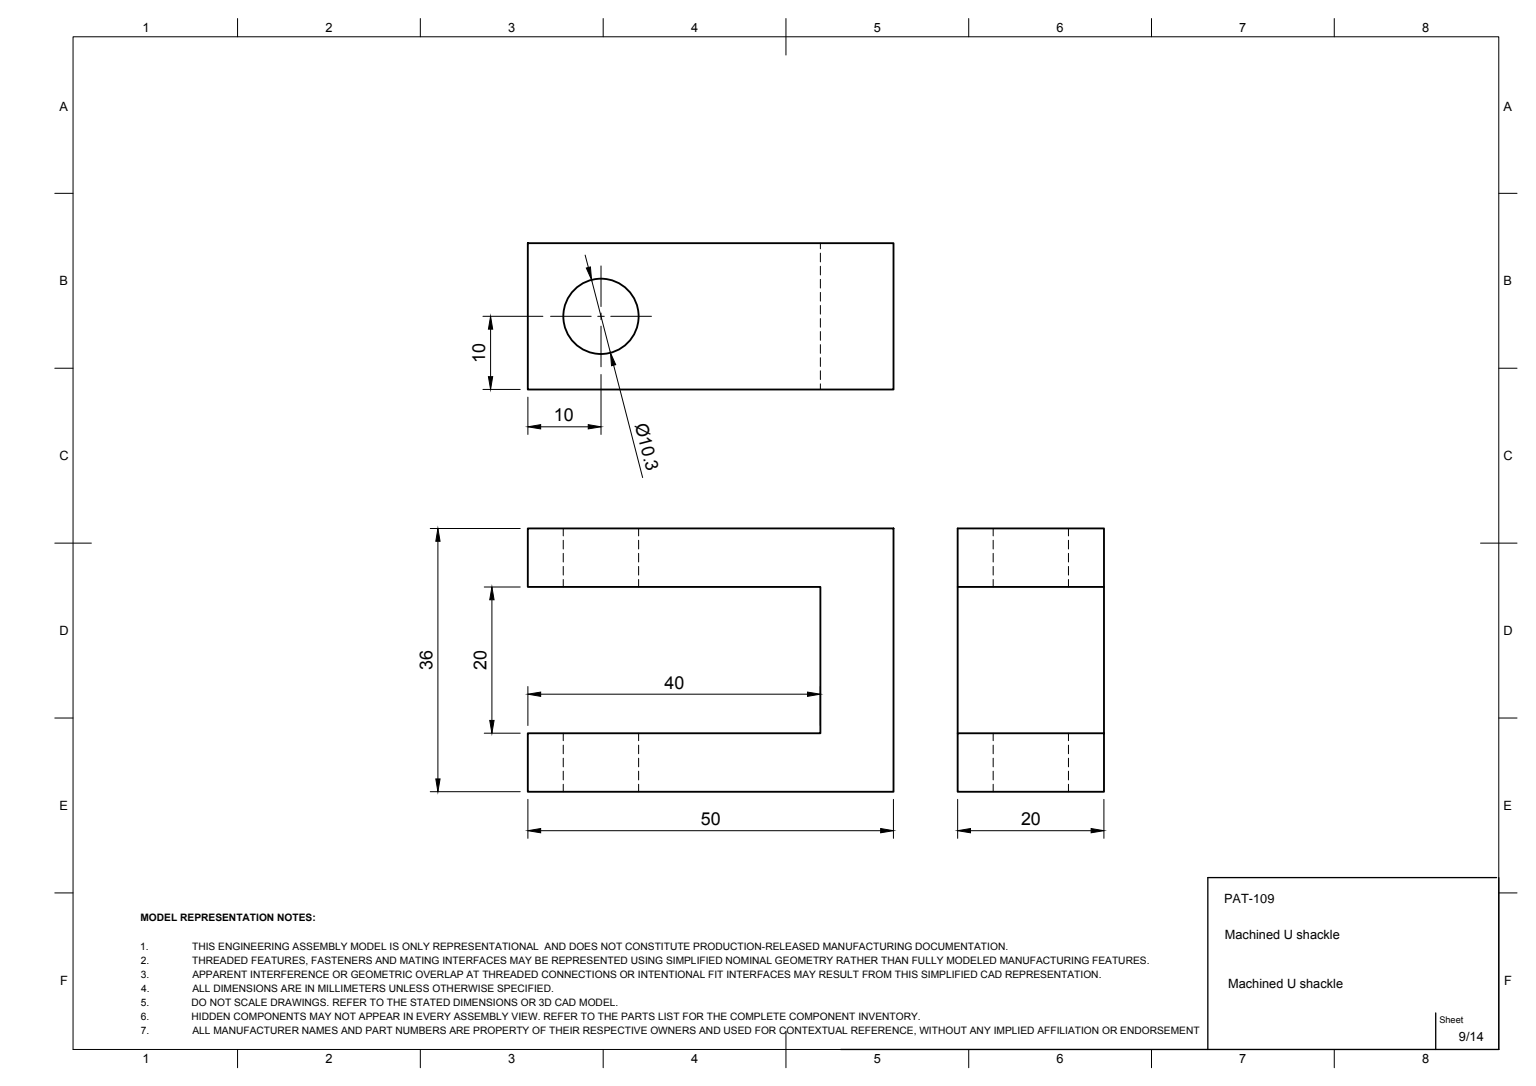
ISO-10303-21;
HEADER;
/* Generated by software containing ST-Developer
 * from STEP Tools, Inc. (www.steptools.com) 
 */

FILE_DESCRIPTION(
/* description */ ('Twin-shackle spreader bar'),
/* implementation_level */ '2;1');

FILE_NAME(
/* name */ 'Machined U shackle.step',
/* time_stamp */ '2026-10-27T20:18:10-07:00',
/* author */ (''),
/* organization */ (''),
/* preprocessor_version */ 'ST-DEVELOPER v20.2',
/* originating_system */ 'Autodesk Translation Framework v15.17.0.0',
/* authorisation */ '');

FILE_SCHEMA (('AUTOMOTIVE_DESIGN { 1 0 10303 214 3 1 1 }'));
ENDSEC;

DATA;
#10=MECHANICAL_DESIGN_GEOMETRIC_PRESENTATION_REPRESENTATION('',(#159),#1829);
#108=CIRCLE('',#1055,0.515000000000001);
#109=CIRCLE('',#1056,0.515000000000001);
#110=CIRCLE('',#1058,0.515000000000001);
#111=CIRCLE('',#1059,0.515000000000001);
#133=CYLINDRICAL_SURFACE('',#1054,0.515000000000001);
#134=CYLINDRICAL_SURFACE('',#1057,0.515000000000001);
#145=SHAPE_REPRESENTATION_RELATIONSHIP('SRR','None',#1883,#152);
#152=ADVANCED_BREP_SHAPE_REPRESENTATION('',(#166),#1824);
#159=STYLED_ITEM('',(#1970),#166);
#166=MANIFOLD_SOLID_BREP('Body1',#939);
#175=FACE_BOUND('',#260,.T.);
#176=FACE_BOUND('',#263,.T.);
#177=FACE_BOUND('',#266,.T.);
#178=FACE_BOUND('',#269,.T.);
#203=FACE_OUTER_BOUND('',#257,.T.);
#204=FACE_OUTER_BOUND('',#258,.T.);
#205=FACE_OUTER_BOUND('',#259,.T.);
#206=FACE_OUTER_BOUND('',#261,.T.);
#207=FACE_OUTER_BOUND('',#262,.T.);
#208=FACE_OUTER_BOUND('',#264,.T.);
#209=FACE_OUTER_BOUND('',#265,.T.);
#210=FACE_OUTER_BOUND('',#267,.T.);
#211=FACE_OUTER_BOUND('',#268,.T.);
#212=FACE_OUTER_BOUND('',#270,.T.);
#213=FACE_OUTER_BOUND('',#271,.T.);
#214=FACE_OUTER_BOUND('',#272,.T.);
#257=EDGE_LOOP('',(#712,#713,#714,#715));
#258=EDGE_LOOP('',(#716,#717,#718,#719));
#259=EDGE_LOOP('',(#720,#721,#722,#723));
#260=EDGE_LOOP('',(#724));
#261=EDGE_LOOP('',(#725,#726,#727,#728));
#262=EDGE_LOOP('',(#729,#730,#731,#732));
#263=EDGE_LOOP('',(#733));
#264=EDGE_LOOP('',(#734,#735,#736,#737));
#265=EDGE_LOOP('',(#738,#739,#740,#741));
#266=EDGE_LOOP('',(#742));
#267=EDGE_LOOP('',(#743,#744,#745,#746));
#268=EDGE_LOOP('',(#747,#748,#749,#750));
#269=EDGE_LOOP('',(#751));
#270=EDGE_LOOP('',(#752,#753,#754,#755));
#271=EDGE_LOOP('',(#756,#757,#758,#759,#760,#761,#762,#763));
#272=EDGE_LOOP('',(#764,#765,#766,#767,#768,#769,#770,#771));
#336=LINE('',#1522,#412);
#337=LINE('',#1528,#413);
#338=LINE('',#1533,#414);
#339=LINE('',#1535,#415);
#340=LINE('',#1537,#416);
#341=LINE('',#1538,#417);
#342=LINE('',#1541,#418);
#343=LINE('',#1543,#419);
#344=LINE('',#1544,#420);
#345=LINE('',#1547,#421);
#346=LINE('',#1549,#422);
#347=LINE('',#1550,#423);
#348=LINE('',#1553,#424);
#349=LINE('',#1555,#425);
#350=LINE('',#1556,#426);
#351=LINE('',#1559,#427);
#352=LINE('',#1561,#428);
#353=LINE('',#1562,#429);
#354=LINE('',#1565,#430);
#355=LINE('',#1567,#431);
#356=LINE('',#1568,#432);
#357=LINE('',#1571,#433);
#358=LINE('',#1573,#434);
#359=LINE('',#1574,#435);
#360=LINE('',#1576,#436);
#361=LINE('',#1577,#437);
#412=VECTOR('',#1234,0.515000000000001);
#413=VECTOR('',#1241,0.515000000000001);
#414=VECTOR('',#1246,1.);
#415=VECTOR('',#1247,1.);
#416=VECTOR('',#1248,1.);
#417=VECTOR('',#1249,1.);
#418=VECTOR('',#1252,1.);
#419=VECTOR('',#1253,1.);
#420=VECTOR('',#1254,1.);
#421=VECTOR('',#1257,1.);
#422=VECTOR('',#1258,1.);
#423=VECTOR('',#1259,1.);
#424=VECTOR('',#1262,1.);
#425=VECTOR('',#1263,1.);
#426=VECTOR('',#1264,1.);
#427=VECTOR('',#1267,1.);
#428=VECTOR('',#1268,1.);
#429=VECTOR('',#1269,1.);
#430=VECTOR('',#1272,1.);
#431=VECTOR('',#1273,1.);
#432=VECTOR('',#1274,1.);
#433=VECTOR('',#1277,1.);
#434=VECTOR('',#1278,1.);
#435=VECTOR('',#1279,1.);
#436=VECTOR('',#1282,1.);
#437=VECTOR('',#1283,1.);
#479=VERTEX_POINT('',#1519);
#480=VERTEX_POINT('',#1521);
#481=VERTEX_POINT('',#1525);
#482=VERTEX_POINT('',#1527);
#483=VERTEX_POINT('',#1531);
#484=VERTEX_POINT('',#1532);
#485=VERTEX_POINT('',#1534);
#486=VERTEX_POINT('',#1536);
#487=VERTEX_POINT('',#1540);
#488=VERTEX_POINT('',#1542);
#489=VERTEX_POINT('',#1546);
#490=VERTEX_POINT('',#1548);
#491=VERTEX_POINT('',#1552);
#492=VERTEX_POINT('',#1554);
#493=VERTEX_POINT('',#1558);
#494=VERTEX_POINT('',#1560);
#495=VERTEX_POINT('',#1564);
#496=VERTEX_POINT('',#1566);
#497=VERTEX_POINT('',#1570);
#498=VERTEX_POINT('',#1572);
#564=EDGE_CURVE('',#479,#479,#108,.T.);
#565=EDGE_CURVE('',#479,#480,#336,.T.);
#566=EDGE_CURVE('',#480,#480,#109,.T.);
#567=EDGE_CURVE('',#481,#481,#110,.T.);
#568=EDGE_CURVE('',#481,#482,#337,.T.);
#569=EDGE_CURVE('',#482,#482,#111,.T.);
#570=EDGE_CURVE('',#483,#484,#338,.T.);
#571=EDGE_CURVE('',#483,#485,#339,.T.);
#572=EDGE_CURVE('',#486,#485,#340,.T.);
#573=EDGE_CURVE('',#484,#486,#341,.T.);
#574=EDGE_CURVE('',#484,#487,#342,.T.);
#575=EDGE_CURVE('',#488,#486,#343,.T.);
#576=EDGE_CURVE('',#487,#488,#344,.T.);
#577=EDGE_CURVE('',#487,#489,#345,.T.);
#578=EDGE_CURVE('',#490,#488,#346,.T.);
#579=EDGE_CURVE('',#489,#490,#347,.T.);
#580=EDGE_CURVE('',#489,#491,#348,.T.);
#581=EDGE_CURVE('',#492,#490,#349,.T.);
#582=EDGE_CURVE('',#491,#492,#350,.T.);
#583=EDGE_CURVE('',#491,#493,#351,.T.);
#584=EDGE_CURVE('',#494,#492,#352,.T.);
#585=EDGE_CURVE('',#493,#494,#353,.T.);
#586=EDGE_CURVE('',#493,#495,#354,.T.);
#587=EDGE_CURVE('',#496,#494,#355,.T.);
#588=EDGE_CURVE('',#495,#496,#356,.T.);
#589=EDGE_CURVE('',#495,#497,#357,.T.);
#590=EDGE_CURVE('',#498,#496,#358,.T.);
#591=EDGE_CURVE('',#497,#498,#359,.T.);
#592=EDGE_CURVE('',#497,#483,#360,.T.);
#593=EDGE_CURVE('',#485,#498,#361,.T.);
#712=ORIENTED_EDGE('',*,*,#564,.F.);
#713=ORIENTED_EDGE('',*,*,#565,.T.);
#714=ORIENTED_EDGE('',*,*,#566,.F.);
#715=ORIENTED_EDGE('',*,*,#565,.F.);
#716=ORIENTED_EDGE('',*,*,#567,.F.);
#717=ORIENTED_EDGE('',*,*,#568,.T.);
#718=ORIENTED_EDGE('',*,*,#569,.F.);
#719=ORIENTED_EDGE('',*,*,#568,.F.);
#720=ORIENTED_EDGE('',*,*,#570,.F.);
#721=ORIENTED_EDGE('',*,*,#571,.T.);
#722=ORIENTED_EDGE('',*,*,#572,.F.);
#723=ORIENTED_EDGE('',*,*,#573,.F.);
#724=ORIENTED_EDGE('',*,*,#567,.T.);
#725=ORIENTED_EDGE('',*,*,#574,.F.);
#726=ORIENTED_EDGE('',*,*,#573,.T.);
#727=ORIENTED_EDGE('',*,*,#575,.F.);
#728=ORIENTED_EDGE('',*,*,#576,.F.);
#729=ORIENTED_EDGE('',*,*,#577,.F.);
#730=ORIENTED_EDGE('',*,*,#576,.T.);
#731=ORIENTED_EDGE('',*,*,#578,.F.);
#732=ORIENTED_EDGE('',*,*,#579,.F.);
#733=ORIENTED_EDGE('',*,*,#569,.T.);
#734=ORIENTED_EDGE('',*,*,#580,.F.);
#735=ORIENTED_EDGE('',*,*,#579,.T.);
#736=ORIENTED_EDGE('',*,*,#581,.F.);
#737=ORIENTED_EDGE('',*,*,#582,.F.);
#738=ORIENTED_EDGE('',*,*,#583,.F.);
#739=ORIENTED_EDGE('',*,*,#582,.T.);
#740=ORIENTED_EDGE('',*,*,#584,.F.);
#741=ORIENTED_EDGE('',*,*,#585,.F.);
#742=ORIENTED_EDGE('',*,*,#564,.T.);
#743=ORIENTED_EDGE('',*,*,#586,.F.);
#744=ORIENTED_EDGE('',*,*,#585,.T.);
#745=ORIENTED_EDGE('',*,*,#587,.F.);
#746=ORIENTED_EDGE('',*,*,#588,.F.);
#747=ORIENTED_EDGE('',*,*,#589,.F.);
#748=ORIENTED_EDGE('',*,*,#588,.T.);
#749=ORIENTED_EDGE('',*,*,#590,.F.);
#750=ORIENTED_EDGE('',*,*,#591,.F.);
#751=ORIENTED_EDGE('',*,*,#566,.T.);
#752=ORIENTED_EDGE('',*,*,#592,.F.);
#753=ORIENTED_EDGE('',*,*,#591,.T.);
#754=ORIENTED_EDGE('',*,*,#593,.F.);
#755=ORIENTED_EDGE('',*,*,#571,.F.);
#756=ORIENTED_EDGE('',*,*,#593,.T.);
#757=ORIENTED_EDGE('',*,*,#590,.T.);
#758=ORIENTED_EDGE('',*,*,#587,.T.);
#759=ORIENTED_EDGE('',*,*,#584,.T.);
#760=ORIENTED_EDGE('',*,*,#581,.T.);
#761=ORIENTED_EDGE('',*,*,#578,.T.);
#762=ORIENTED_EDGE('',*,*,#575,.T.);
#763=ORIENTED_EDGE('',*,*,#572,.T.);
#764=ORIENTED_EDGE('',*,*,#592,.T.);
#765=ORIENTED_EDGE('',*,*,#570,.T.);
#766=ORIENTED_EDGE('',*,*,#574,.T.);
#767=ORIENTED_EDGE('',*,*,#577,.T.);
#768=ORIENTED_EDGE('',*,*,#580,.T.);
#769=ORIENTED_EDGE('',*,*,#583,.T.);
#770=ORIENTED_EDGE('',*,*,#586,.T.);
#771=ORIENTED_EDGE('',*,*,#589,.T.);
#867=PLANE('',#1060);
#868=PLANE('',#1061);
#869=PLANE('',#1062);
#870=PLANE('',#1063);
#871=PLANE('',#1064);
#872=PLANE('',#1065);
#873=PLANE('',#1066);
#874=PLANE('',#1067);
#875=PLANE('',#1068);
#876=PLANE('',#1069);
#904=ADVANCED_FACE('',(#203),#133,.F.);
#905=ADVANCED_FACE('',(#204),#134,.F.);
#906=ADVANCED_FACE('',(#205,#175),#867,.T.);
#907=ADVANCED_FACE('',(#206),#868,.T.);
#908=ADVANCED_FACE('',(#207,#176),#869,.T.);
#909=ADVANCED_FACE('',(#208),#870,.T.);
#910=ADVANCED_FACE('',(#209,#177),#871,.T.);
#911=ADVANCED_FACE('',(#210),#872,.T.);
#912=ADVANCED_FACE('',(#211,#178),#873,.T.);
#913=ADVANCED_FACE('',(#212),#874,.T.);
#914=ADVANCED_FACE('',(#213),#875,.T.);
#915=ADVANCED_FACE('',(#214),#876,.F.);
#939=CLOSED_SHELL('',(#904,#905,#906,#907,#908,#909,#910,#911,#912,#913,
#914,#915));
#1053=AXIS2_PLACEMENT_3D('',#1517,#1228,#1229);
#1054=AXIS2_PLACEMENT_3D('',#1518,#1230,#1231);
#1055=AXIS2_PLACEMENT_3D('',#1520,#1232,#1233);
#1056=AXIS2_PLACEMENT_3D('',#1523,#1235,#1236);
#1057=AXIS2_PLACEMENT_3D('',#1524,#1237,#1238);
#1058=AXIS2_PLACEMENT_3D('',#1526,#1239,#1240);
#1059=AXIS2_PLACEMENT_3D('',#1529,#1242,#1243);
#1060=AXIS2_PLACEMENT_3D('',#1530,#1244,#1245);
#1061=AXIS2_PLACEMENT_3D('',#1539,#1250,#1251);
#1062=AXIS2_PLACEMENT_3D('',#1545,#1255,#1256);
#1063=AXIS2_PLACEMENT_3D('',#1551,#1260,#1261);
#1064=AXIS2_PLACEMENT_3D('',#1557,#1265,#1266);
#1065=AXIS2_PLACEMENT_3D('',#1563,#1270,#1271);
#1066=AXIS2_PLACEMENT_3D('',#1569,#1275,#1276);
#1067=AXIS2_PLACEMENT_3D('',#1575,#1280,#1281);
#1068=AXIS2_PLACEMENT_3D('',#1578,#1284,#1285);
#1069=AXIS2_PLACEMENT_3D('',#1579,#1286,#1287);
#1228=DIRECTION('axis',(0.,0.,1.));
#1229=DIRECTION('refdir',(1.,0.,0.));
#1230=DIRECTION('center_axis',(0.,1.,0.));
#1231=DIRECTION('ref_axis',(1.,0.,0.));
#1232=DIRECTION('center_axis',(0.,1.,0.));
#1233=DIRECTION('ref_axis',(1.,0.,0.));
#1234=DIRECTION('',(0.,1.,0.));
#1235=DIRECTION('center_axis',(0.,-1.,0.));
#1236=DIRECTION('ref_axis',(1.,0.,0.));
#1237=DIRECTION('center_axis',(0.,1.,0.));
#1238=DIRECTION('ref_axis',(1.,0.,0.));
#1239=DIRECTION('center_axis',(0.,1.,0.));
#1240=DIRECTION('ref_axis',(1.,0.,0.));
#1241=DIRECTION('',(0.,1.,0.));
#1242=DIRECTION('center_axis',(0.,-1.,0.));
#1243=DIRECTION('ref_axis',(1.,0.,0.));
#1244=DIRECTION('center_axis',(0.,-1.,0.));
#1245=DIRECTION('ref_axis',(0.,0.,-1.));
#1246=DIRECTION('',(0.,0.,1.));
#1247=DIRECTION('',(1.,0.,0.));
#1248=DIRECTION('',(0.,0.,-1.));
#1249=DIRECTION('',(1.,0.,0.));
#1250=DIRECTION('center_axis',(0.,0.,1.));
#1251=DIRECTION('ref_axis',(0.,-1.,0.));
#1252=DIRECTION('',(0.,1.,0.));
#1253=DIRECTION('',(0.,-1.,0.));
#1254=DIRECTION('',(1.,0.,0.));
#1255=DIRECTION('center_axis',(0.,1.,0.));
#1256=DIRECTION('ref_axis',(0.,0.,1.));
#1257=DIRECTION('',(0.,0.,-1.));
#1258=DIRECTION('',(0.,0.,1.));
#1259=DIRECTION('',(1.,0.,0.));
#1260=DIRECTION('center_axis',(0.,0.,1.));
#1261=DIRECTION('ref_axis',(0.,-1.,0.));
#1262=DIRECTION('',(0.,1.,0.));
#1263=DIRECTION('',(0.,-1.,0.));
#1264=DIRECTION('',(1.,0.,0.));
#1265=DIRECTION('center_axis',(0.,-1.,0.));
#1266=DIRECTION('ref_axis',(0.,0.,-1.));
#1267=DIRECTION('',(0.,0.,1.));
#1268=DIRECTION('',(0.,0.,-1.));
#1269=DIRECTION('',(1.,0.,0.));
#1270=DIRECTION('center_axis',(0.,0.,1.));
#1271=DIRECTION('ref_axis',(0.,-1.,0.));
#1272=DIRECTION('',(0.,1.,0.));
#1273=DIRECTION('',(0.,-1.,0.));
#1274=DIRECTION('',(1.,0.,0.));
#1275=DIRECTION('center_axis',(0.,1.,0.));
#1276=DIRECTION('ref_axis',(0.,0.,1.));
#1277=DIRECTION('',(0.,0.,-1.));
#1278=DIRECTION('',(0.,0.,1.));
#1279=DIRECTION('',(1.,0.,0.));
#1280=DIRECTION('center_axis',(0.,0.,-1.));
#1281=DIRECTION('ref_axis',(0.,1.,0.));
#1282=DIRECTION('',(0.,-1.,0.));
#1283=DIRECTION('',(0.,1.,0.));
#1284=DIRECTION('center_axis',(1.,0.,0.));
#1285=DIRECTION('ref_axis',(0.,0.,-1.));
#1286=DIRECTION('center_axis',(1.,0.,0.));
#1287=DIRECTION('ref_axis',(0.,0.,-1.));
#1517=CARTESIAN_POINT('',(0.,0.,0.));
#1518=CARTESIAN_POINT('Origin',(-21.,-1.9,-2.));
#1519=CARTESIAN_POINT('',(-21.515,1.,-2.));
#1520=CARTESIAN_POINT('Origin',(-21.,1.,-2.));
#1521=CARTESIAN_POINT('',(-21.515,1.8,-2.));
#1522=CARTESIAN_POINT('',(-21.515,-1.9,-2.));
#1523=CARTESIAN_POINT('Origin',(-21.,1.8,-2.));
#1524=CARTESIAN_POINT('Origin',(-21.,-1.9,-2.));
#1525=CARTESIAN_POINT('',(-21.515,-1.8,-2.));
#1526=CARTESIAN_POINT('Origin',(-21.,-1.8,-2.));
#1527=CARTESIAN_POINT('',(-21.515,-1.,-2.));
#1528=CARTESIAN_POINT('',(-21.515,-1.9,-2.));
#1529=CARTESIAN_POINT('Origin',(-21.,-1.,-2.));
#1530=CARTESIAN_POINT('Origin',(-22.,-1.8,-1.));
#1531=CARTESIAN_POINT('',(-22.,-1.8,-6.));
#1532=CARTESIAN_POINT('',(-22.,-1.8,-1.));
#1533=CARTESIAN_POINT('',(-22.,-1.8,-6.));
#1534=CARTESIAN_POINT('',(-20.,-1.8,-6.));
#1535=CARTESIAN_POINT('',(-22.,-1.8,-6.));
#1536=CARTESIAN_POINT('',(-20.,-1.8,-1.));
#1537=CARTESIAN_POINT('',(-20.,-1.8,-6.));
#1538=CARTESIAN_POINT('',(-22.,-1.8,-1.));
#1539=CARTESIAN_POINT('Origin',(-22.,-1.,-1.));
#1540=CARTESIAN_POINT('',(-22.,-1.,-1.));
#1541=CARTESIAN_POINT('',(-22.,-1.8,-1.));
#1542=CARTESIAN_POINT('',(-20.,-1.,-1.));
#1543=CARTESIAN_POINT('',(-20.,-1.8,-1.));
#1544=CARTESIAN_POINT('',(-22.,-1.,-1.));
#1545=CARTESIAN_POINT('Origin',(-22.,-1.,-5.));
#1546=CARTESIAN_POINT('',(-22.,-1.,-5.));
#1547=CARTESIAN_POINT('',(-22.,-1.,-1.));
#1548=CARTESIAN_POINT('',(-20.,-1.,-5.));
#1549=CARTESIAN_POINT('',(-20.,-1.,-1.));
#1550=CARTESIAN_POINT('',(-22.,-1.,-5.));
#1551=CARTESIAN_POINT('Origin',(-22.,1.,-5.));
#1552=CARTESIAN_POINT('',(-22.,1.,-5.));
#1553=CARTESIAN_POINT('',(-22.,-1.,-5.));
#1554=CARTESIAN_POINT('',(-20.,1.,-5.));
#1555=CARTESIAN_POINT('',(-20.,-1.,-5.));
#1556=CARTESIAN_POINT('',(-22.,1.,-5.));
#1557=CARTESIAN_POINT('Origin',(-22.,1.,-1.));
#1558=CARTESIAN_POINT('',(-22.,1.,-1.));
#1559=CARTESIAN_POINT('',(-22.,1.,-5.));
#1560=CARTESIAN_POINT('',(-20.,1.,-1.));
#1561=CARTESIAN_POINT('',(-20.,1.,-5.));
#1562=CARTESIAN_POINT('',(-22.,1.,-1.));
#1563=CARTESIAN_POINT('Origin',(-22.,1.8,-1.));
#1564=CARTESIAN_POINT('',(-22.,1.8,-1.));
#1565=CARTESIAN_POINT('',(-22.,1.,-1.));
#1566=CARTESIAN_POINT('',(-20.,1.8,-1.));
#1567=CARTESIAN_POINT('',(-20.,1.,-1.));
#1568=CARTESIAN_POINT('',(-22.,1.8,-1.));
#1569=CARTESIAN_POINT('Origin',(-22.,1.8,-6.));
#1570=CARTESIAN_POINT('',(-22.,1.8,-6.));
#1571=CARTESIAN_POINT('',(-22.,1.8,-1.));
#1572=CARTESIAN_POINT('',(-20.,1.8,-6.));
#1573=CARTESIAN_POINT('',(-20.,1.8,-1.));
#1574=CARTESIAN_POINT('',(-22.,1.8,-6.));
#1575=CARTESIAN_POINT('Origin',(-22.,-1.8,-6.));
#1576=CARTESIAN_POINT('',(-22.,1.8,-6.));
#1577=CARTESIAN_POINT('',(-20.,1.8,-6.));
#1578=CARTESIAN_POINT('Origin',(-20.,0.,-3.5));
#1579=CARTESIAN_POINT('Origin',(-22.,0.,-3.5));
#1812=UNCERTAINTY_MEASURE_WITH_UNIT(LENGTH_MEASURE(0.001),#1830,
'DISTANCE_ACCURACY_VALUE',
'Maximum model space distance between geometric entities at asserted c
onnectivities');
#1817=UNCERTAINTY_MEASURE_WITH_UNIT(LENGTH_MEASURE(0.001),#1830,
'DISTANCE_ACCURACY_VALUE',
'Maximum model space distance between geometric entities at asserted c
onnectivities');
#1824=(
GEOMETRIC_REPRESENTATION_CONTEXT(3)
GLOBAL_UNCERTAINTY_ASSIGNED_CONTEXT((#1812))
GLOBAL_UNIT_ASSIGNED_CONTEXT((#1830,#1832,#1833))
REPRESENTATION_CONTEXT('','3D')
);
#1829=(
GEOMETRIC_REPRESENTATION_CONTEXT(3)
GLOBAL_UNCERTAINTY_ASSIGNED_CONTEXT((#1817))
GLOBAL_UNIT_ASSIGNED_CONTEXT((#1830,#1832,#1833))
REPRESENTATION_CONTEXT('','3D')
);
#1830=(
LENGTH_UNIT()
NAMED_UNIT(*)
SI_UNIT(.CENTI.,.METRE.)
);
#1832=(
NAMED_UNIT(*)
PLANE_ANGLE_UNIT()
SI_UNIT($,.RADIAN.)
);
#1833=(
NAMED_UNIT(*)
SI_UNIT($,.STERADIAN.)
SOLID_ANGLE_UNIT()
);
#1840=SHAPE_DEFINITION_REPRESENTATION(#1855,#1883);
#1855=PRODUCT_DEFINITION_SHAPE('',$,#1895);
#1883=SHAPE_REPRESENTATION('',(#1053),#1824);
#1888=PRODUCT_DEFINITION_CONTEXT('part definition',#1923,'design');
#1895=PRODUCT_DEFINITION('Machined U shackle','Machined U shackle',#1906,
#1888);
#1906=PRODUCT_DEFINITION_FORMATION('',$,#1931);
#1923=APPLICATION_CONTEXT(
'Core Data for Automotive Mechanical Design Process');
#1924=PRODUCT_CONTEXT('part definition',#1923,'mechanical');
#1931=PRODUCT('Machined U shackle','Machined U shackle',
'Machined U shackle',(#1924));
#1964=COLOUR_RGB('Light Blue',0.38,0.62,0.78);
#1965=FILL_AREA_STYLE_COLOUR('',#1964);
#1966=FILL_AREA_STYLE('',(#1965));
#1967=SURFACE_STYLE_FILL_AREA(#1966);
#1968=SURFACE_SIDE_STYLE('',(#1967));
#1969=SURFACE_STYLE_USAGE(.BOTH.,#1968);
#1970=PRESENTATION_STYLE_ASSIGNMENT((#1969));
ENDSEC;
END-ISO-10303-21;
